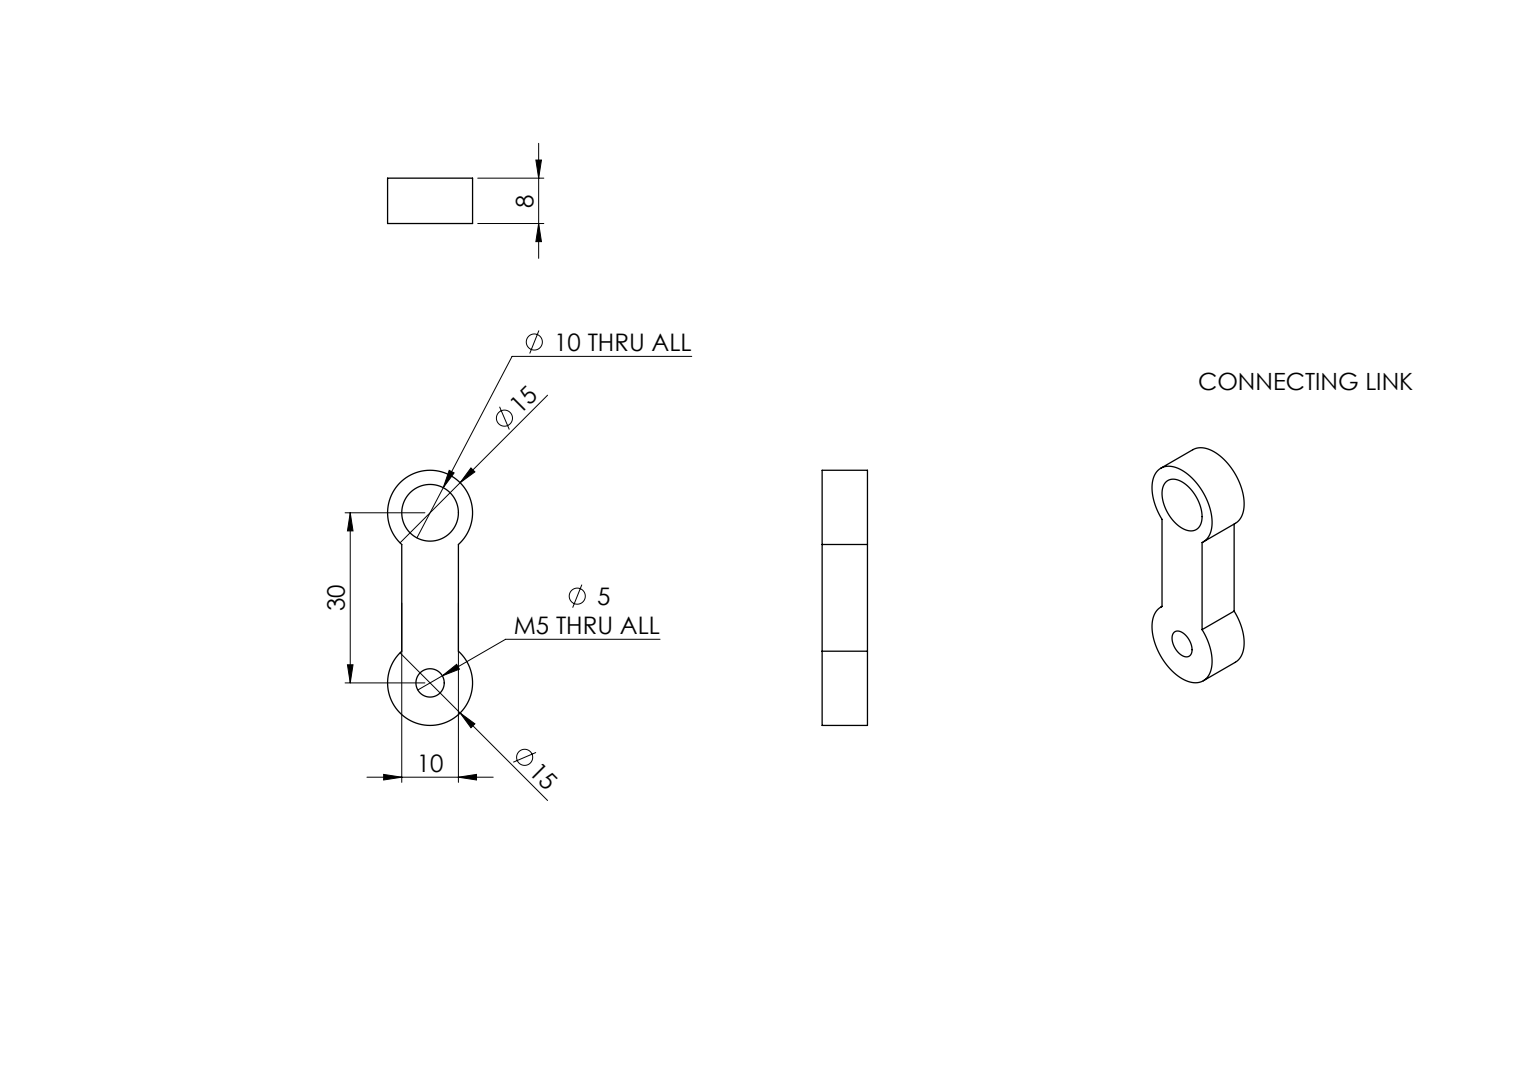
ISO-10303-21;
HEADER;
FILE_DESCRIPTION (('STEP AP214'),
    '1' );
FILE_NAME ('connecting link.step',
    '2026-10-25T11:00:22',
    ( '' ),
    ( '' ),
    'SwSTEP 2.0',
    'SolidWorks 2026',
    '' );
FILE_SCHEMA (( 'AUTOMOTIVE_DESIGN' ));
ENDSEC;

DATA;
#10=DIRECTION ( 'NONE',  ( -1.000000000000000000, 0.000000000000000000, 0.000000000000000000 ) ) ;
#19=CARTESIAN_POINT ( 'NONE',  ( -5.000000000000000000, 5.590169943749474513, 10.00000000000000000 ) ) ;
#25=CYLINDRICAL_SURFACE ( 'NONE', #3173, 4.999999999999999112 ) ;
#27=DIRECTION ( 'NONE',  ( -0.000000000000000000, -0.000000000000000000, -1.000000000000000000 ) ) ;
#30=( LENGTH_UNIT ( ) NAMED_UNIT ( * ) SI_UNIT ( .MILLI., .METRE. ) );
#32=DIRECTION ( 'NONE',  ( -0.000000000000000000, -0.000000000000000000, -1.000000000000000000 ) ) ;
#36=EDGE_CURVE ( 'NONE', #2171, #1853, #1673, .T. ) ;
#37=CIRCLE ( 'NONE', #1306, 7.500000000000000000 ) ;
#58=ORIENTED_EDGE ( 'NONE', *, *, #3093, .T. ) ;
#60=CARTESIAN_POINT ( 'NONE',  ( 4.999999999999999112, 30.00000000000000000, 18.00000000000000355 ) ) ;
#71=CARTESIAN_POINT ( 'NONE',  ( -7.500000000000000000, 0.000000000000000000, 10.00000000000000000 ) ) ;
#73=CARTESIAN_POINT ( 'NONE',  ( 5.000000000000000000, 24.40983005625052726, 18.00000000000000355 ) ) ;
#75=( LENGTH_UNIT ( ) NAMED_UNIT ( * ) SI_UNIT ( .MILLI., .METRE. ) );
#88=ORIENTED_EDGE ( 'NONE', *, *, #36, .T. ) ;
#95=DIRECTION ( 'NONE',  ( -0.000000000000000000, 0.000000000000000000, 1.000000000000000000 ) ) ;
#106=AXIS2_PLACEMENT_3D ( 'NONE', #3179, #664, #3192 ) ;
#113=DIRECTION ( 'NONE',  ( 1.000000000000000000, 0.000000000000000000, 0.000000000000000000 ) ) ;
#125=ORIENTED_EDGE ( 'NONE', *, *, #751, .F. ) ;
#136=EDGE_CURVE ( 'NONE', #870, #2195, #2997, .T. ) ;
#138=AXIS2_PLACEMENT_3D ( 'NONE', #166, #181, #437 ) ;
#146=DIRECTION ( 'NONE',  ( -0.000000000000000000, -0.000000000000000000, -1.000000000000000000 ) ) ;
#152=AXIS2_PLACEMENT_3D ( 'NONE', #2297, #2784, #10 ) ;
#153=CYLINDRICAL_SURFACE ( 'NONE', #3180, 2.499999999999999556 ) ;
#161=EDGE_CURVE ( 'NONE', #1969, #1853, #1067, .T. ) ;
#166=CARTESIAN_POINT ( 'NONE',  ( 0.000000000000000000, 30.00000000000000000, 18.00000000000000355 ) ) ;
#181=DIRECTION ( 'NONE',  ( -0.000000000000000000, -0.000000000000000000, -1.000000000000000000 ) ) ;
#199=ORIENTED_EDGE ( 'NONE', *, *, #2749, .T. ) ;
#207=DIRECTION ( 'NONE',  ( 1.000000000000000000, 0.000000000000000000, 0.000000000000000000 ) ) ;
#222=DIRECTION ( 'NONE',  ( -0.000000000000000000, -0.000000000000000000, -1.000000000000000000 ) ) ;
#237=DIRECTION ( 'NONE',  ( 0.000000000000000000, 0.000000000000000000, 1.000000000000000000 ) ) ;
#243=CIRCLE ( 'NONE', #1828, 7.500000000000000888 ) ;
#245=VECTOR ( 'NONE', #2046, 1000.000000000000000 ) ;
#247=ORIENTED_EDGE ( 'NONE', *, *, #1457, .T. ) ;
#248=AXIS2_PLACEMENT_3D ( 'NONE', #2084, #843, #1137 ) ;
#252=CARTESIAN_POINT ( 'NONE',  ( 0.000000000000000000, 0.000000000000000000, 18.00000000000000355 ) ) ;
#256=SURFACE_SIDE_STYLE ('',( #1538 ) ) ;
#271=FACE_OUTER_BOUND ( 'NONE', #2659, .T. ) ;
#278=( NAMED_UNIT ( * ) PLANE_ANGLE_UNIT ( ) SI_UNIT ( $, .RADIAN. ) );
#280=ADVANCED_FACE ( 'NONE', ( #1859 ), #1120, .F. ) ;
#282=CARTESIAN_POINT ( 'NONE',  ( -7.500000000000000888, 30.00000000000000000, 18.00000000000000355 ) ) ;
#283=ORIENTED_EDGE ( 'NONE', *, *, #618, .F. ) ;
#300=ORIENTED_EDGE ( 'NONE', *, *, #804, .T. ) ;
#303=EDGE_CURVE ( 'NONE', #1969, #1046, #611, .T. ) ;
#310=CARTESIAN_POINT ( 'NONE',  ( 5.000000000000000000, 5.590169943749473624, 10.00000000000000178 ) ) ;
#312=EDGE_LOOP ( 'NONE', ( #1653, #125 ) ) ;
#313=LINE ( 'NONE', #1936, #1957 ) ;
#314=AXIS2_PLACEMENT_3D ( 'NONE', #858, #1399, #2660 ) ;
#317=ORIENTED_EDGE ( 'NONE', *, *, #2514, .F. ) ;
#327=FILL_AREA_STYLE ('',( #2835 ) ) ;
#334=CARTESIAN_POINT ( 'NONE',  ( -4.999999999999999112, 30.00000000000000000, 18.00000000000000355 ) ) ;
#338=ORIENTED_EDGE ( 'NONE', *, *, #2208, .F. ) ;
#342=VERTEX_POINT ( 'NONE', #19 ) ;
#347=EDGE_CURVE ( 'NONE', #1810, #870, #2221, .T. ) ;
#352=EDGE_LOOP ( 'NONE', ( #2643, #317, #2086, #589 ) ) ;
#357=PRODUCT ( 'connecting link', 'connecting link', '', ( #2766 ) ) ;
#362=EDGE_CURVE ( 'NONE', #342, #3130, #37, .T. ) ;
#371=AXIS2_PLACEMENT_3D ( 'NONE', #462, #759, #1502 ) ;
#376=ORIENTED_EDGE ( 'NONE', *, *, #347, .F. ) ;
#380=ORIENTED_EDGE ( 'NONE', *, *, #362, .T. ) ;
#409=ORIENTED_EDGE ( 'NONE', *, *, #362, .F. ) ;
#431=MECHANICAL_DESIGN_GEOMETRIC_PRESENTATION_REPRESENTATION('',(#1645),#485);
#437=DIRECTION ( 'NONE',  ( -1.000000000000000000, 0.000000000000000000, 0.000000000000000000 ) ) ;
#439=VERTEX_POINT ( 'NONE', #282 ) ;
#445=DIRECTION ( 'NONE',  ( 1.000000000000000000, 0.000000000000000000, 0.000000000000000000 ) ) ;
#447=CARTESIAN_POINT ( 'NONE',  ( -2.499999999999999556, 3.061616997868382648E-16, 10.00000000000000000 ) ) ;
#462=CARTESIAN_POINT ( 'NONE',  ( 0.000000000000000000, 30.00000000000000000, 18.00000000000000355 ) ) ;
#464=EDGE_CURVE ( 'NONE', #1883, #2883, #2843, .T. ) ;
#469=CARTESIAN_POINT ( 'NONE',  ( 0.000000000000000000, 30.00000000000000000, 18.00000000000000355 ) ) ;
#475=CARTESIAN_POINT ( 'NONE',  ( 0.000000000000000000, 30.00000000000000000, 10.00000000000000000 ) ) ;
#478=DIRECTION ( 'NONE',  ( 1.000000000000000000, 0.000000000000000000, 0.000000000000000000 ) ) ;
#485=( GEOMETRIC_REPRESENTATION_CONTEXT ( 3 ) GLOBAL_UNCERTAINTY_ASSIGNED_CONTEXT ( ( #770 ) ) GLOBAL_UNIT_ASSIGNED_CONTEXT ( ( #75, #3051, #1811 ) ) REPRESENTATION_CONTEXT ( 'NONE', 'WORKASPACE' ) );
#488=ORIENTED_EDGE ( 'NONE', *, *, #2125, .F. ) ;
#500=EDGE_LOOP ( 'NONE', ( #2350, #616 ) ) ;
#508=LINE ( 'NONE', #2045, #3059 ) ;
#520=EDGE_LOOP ( 'NONE', ( #2673, #606, #711, #2356 ) ) ;
#548=LINE ( 'NONE', #2266, #1038 ) ;
#558=EDGE_CURVE ( 'NONE', #1156, #900, #2476, .T. ) ;
#560=ORIENTED_EDGE ( 'NONE', *, *, #1874, .F. ) ;
#561=DIRECTION ( 'NONE',  ( 1.000000000000000000, 0.000000000000000000, 0.000000000000000000 ) ) ;
#563=EDGE_LOOP ( 'NONE', ( #962, #2420, #624, #283 ) ) ;
#567=ORIENTED_EDGE ( 'NONE', *, *, #2749, .F. ) ;
#576=EDGE_LOOP ( 'NONE', ( #2530, #2251, #199, #247, #1827, #3157, #1316, #88 ) ) ;
#578=CARTESIAN_POINT ( 'NONE',  ( 0.000000000000000000, 30.00000000000000000, 18.00000000000000355 ) ) ;
#582=ORIENTED_EDGE ( 'NONE', *, *, #2260, .F. ) ;
#583=AXIS2_PLACEMENT_3D ( 'NONE', #2757, #3243, #478 ) ;
#585=VECTOR ( 'NONE', #739, 1000.000000000000000 ) ;
#589=ORIENTED_EDGE ( 'NONE', *, *, #2208, .T. ) ;
#595=CARTESIAN_POINT ( 'NONE',  ( 0.000000000000000000, 0.000000000000000000, 10.00000000000000000 ) ) ;
#599=DIRECTION ( 'NONE',  ( -1.000000000000000000, 0.000000000000000000, -0.000000000000000000 ) ) ;
#606=ORIENTED_EDGE ( 'NONE', *, *, #161, .T. ) ;
#611=LINE ( 'NONE', #73, #1572 ) ;
#616=ORIENTED_EDGE ( 'NONE', *, *, #136, .F. ) ;
#617=ADVANCED_BREP_SHAPE_REPRESENTATION ( '', ( #1595, #1692 ), #2651 ) ;
#618=EDGE_CURVE ( 'NONE', #1320, #3085, #548, .T. ) ;
#624=ORIENTED_EDGE ( 'NONE', *, *, #2822, .T. ) ;
#630=VECTOR ( 'NONE', #32, 1000.000000000000000 ) ;
#631=ORIENTED_EDGE ( 'NONE', *, *, #2234, .F. ) ;
#636=ADVANCED_FACE ( 'NONE', ( #1251 ), #2803, .F. ) ;
#642=AXIS2_PLACEMENT_3D ( 'NONE', #1934, #2512, #954 ) ;
#652=ADVANCED_FACE ( 'NONE', ( #1812, #1779, #2515 ), #3022, .T. ) ;
#664=DIRECTION ( 'NONE',  ( -0.000000000000000000, -0.000000000000000000, 1.000000000000000000 ) ) ;
#670=DIRECTION ( 'NONE',  ( 0.000000000000000000, 0.000000000000000000, 1.000000000000000000 ) ) ;
#676=DIRECTION ( 'NONE',  ( -0.000000000000000000, -0.000000000000000000, -1.000000000000000000 ) ) ;
#694=VERTEX_POINT ( 'NONE', #2035 ) ;
#696=CARTESIAN_POINT ( 'NONE',  ( 0.000000000000000000, 30.00000000000000000, 18.00000000000000355 ) ) ;
#699=LINE ( 'NONE', #985, #1260 ) ;
#708=CARTESIAN_POINT ( 'NONE',  ( 0.000000000000000000, 30.00000000000000000, 18.00000000000000355 ) ) ;
#711=ORIENTED_EDGE ( 'NONE', *, *, #1884, .T. ) ;
#716=DIRECTION ( 'NONE',  ( -1.000000000000000000, 0.000000000000000000, 0.000000000000000000 ) ) ;
#723=DIRECTION ( 'NONE',  ( -0.000000000000000000, -0.000000000000000000, -1.000000000000000000 ) ) ;
#725=DIRECTION ( 'NONE',  ( 1.000000000000000000, 0.000000000000000000, 0.000000000000000000 ) ) ;
#737=ORIENTED_EDGE ( 'NONE', *, *, #2840, .T. ) ;
#739=DIRECTION ( 'NONE',  ( -0.000000000000000000, -0.000000000000000000, 1.000000000000000000 ) ) ;
#742=CIRCLE ( 'NONE', #2590, 2.499999999999999556 ) ;
#743=FACE_BOUND ( 'NONE', #2335, .T. ) ;
#751=EDGE_CURVE ( 'NONE', #2182, #2708, #3107, .T. ) ;
#753=ORIENTED_EDGE ( 'NONE', *, *, #2111, .F. ) ;
#759=DIRECTION ( 'NONE',  ( 0.000000000000000000, 0.000000000000000000, 1.000000000000000000 ) ) ;
#768=CARTESIAN_POINT ( 'NONE',  ( 0.000000000000000000, 0.000000000000000000, 18.00000000000000355 ) ) ;
#770=UNCERTAINTY_MEASURE_WITH_UNIT (LENGTH_MEASURE( 1.000000000000000082E-05 ), #75, 'distance_accuracy_value', 'NONE');
#781=DIRECTION ( 'NONE',  ( -0.000000000000000000, -0.000000000000000000, 1.000000000000000000 ) ) ;
#789=DIRECTION ( 'NONE',  ( -0.000000000000000000, -0.000000000000000000, 1.000000000000000000 ) ) ;
#790=CARTESIAN_POINT ( 'NONE',  ( 0.000000000000000000, 30.00000000000000000, 18.00000000000000355 ) ) ;
#799=ORIENTED_EDGE ( 'NONE', *, *, #2840, .F. ) ;
#804=EDGE_CURVE ( 'NONE', #694, #2199, #2047, .T. ) ;
#808=DIRECTION ( 'NONE',  ( 1.000000000000000000, 0.000000000000000000, -0.000000000000000000 ) ) ;
#837=EDGE_CURVE ( 'NONE', #2412, #2195, #3144, .T. ) ;
#843=DIRECTION ( 'NONE',  ( -0.000000000000000000, -0.000000000000000000, 1.000000000000000000 ) ) ;
#847=CARTESIAN_POINT ( 'NONE',  ( -4.999999999999998224, 30.00000000000000000, 10.00000000000000000 ) ) ;
#856=PRODUCT_DEFINITION_FORMATION_WITH_SPECIFIED_SOURCE ( 'ANY', '', #357, .NOT_KNOWN. ) ;
#858=CARTESIAN_POINT ( 'NONE',  ( 0.000000000000000000, 30.00000000000000000, 10.00000000000000000 ) ) ;
#859=DIRECTION ( 'NONE',  ( 1.000000000000000000, 0.000000000000000000, 0.000000000000000000 ) ) ;
#865=ORIENTED_EDGE ( 'NONE', *, *, #2062, .F. ) ;
#870=VERTEX_POINT ( 'NONE', #2333 ) ;
#878=ORIENTED_EDGE ( 'NONE', *, *, #2178, .F. ) ;
#886=PRODUCT_DEFINITION_SHAPE ( 'NONE', 'NONE',  #3057 ) ;
#893=ORIENTED_EDGE ( 'NONE', *, *, #2988, .F. ) ;
#900=VERTEX_POINT ( 'NONE', #310 ) ;
#915=DIRECTION ( 'NONE',  ( -1.000000000000000000, 0.000000000000000000, 0.000000000000000000 ) ) ;
#928=ORIENTED_EDGE ( 'NONE', *, *, #837, .T. ) ;
#933=EDGE_LOOP ( 'NONE', ( #1125, #878, #1413, #2404 ) ) ;
#934=DIRECTION ( 'NONE',  ( 1.000000000000000000, 0.000000000000000000, 0.000000000000000000 ) ) ;
#945=AXIS2_PLACEMENT_3D ( 'NONE', #2977, #2731, #716 ) ;
#949=ORIENTED_EDGE ( 'NONE', *, *, #2612, .T. ) ;
#951=CARTESIAN_POINT ( 'NONE',  ( -5.000000000000000000, 30.00000000000000000, 10.00000000000000178 ) ) ;
#954=DIRECTION ( 'NONE',  ( 1.000000000000000000, 0.000000000000000000, 0.000000000000000000 ) ) ;
#962=ORIENTED_EDGE ( 'NONE', *, *, #1457, .F. ) ;
#970=LINE ( 'NONE', #1953, #1479 ) ;
#978=ADVANCED_FACE ( 'NONE', ( #3108 ), #2402, .T. ) ;
#982=STYLED_ITEM('',(#3300),#1595);
#985=CARTESIAN_POINT ( 'NONE',  ( 5.000000000000000000, 30.00000000000000000, 10.00000000000000178 ) ) ;
#989=DIRECTION ( 'NONE',  ( -1.000000000000000000, 0.000000000000000000, -0.000000000000000000 ) ) ;
#997=CARTESIAN_POINT ( 'NONE',  ( -7.500000000000000000, 0.000000000000000000, 18.00000000000000355 ) ) ;
#1001=PRODUCT_DEFINITION_CONTEXT ( 'detailed design', #2486, 'design' ) ;
#1009=ORIENTED_EDGE ( 'NONE', *, *, #2612, .F. ) ;
#1016=CARTESIAN_POINT ( 'NONE',  ( -5.000000000000000000, 5.590169943749474513, 18.00000000000000355 ) ) ;
#1022=CARTESIAN_POINT ( 'NONE',  ( -5.000000000000000000, 5.590169943749473624, 18.00000000000000355 ) ) ;
#1025=DIRECTION ( 'NONE',  ( -0.000000000000000000, -0.000000000000000000, 1.000000000000000000 ) ) ;
#1030=FACE_OUTER_BOUND ( 'NONE', #1593, .T. ) ;
#1031=CARTESIAN_POINT ( 'NONE',  ( 0.000000000000000000, 30.00000000000000000, 18.00000000000000355 ) ) ;
#1032=CARTESIAN_POINT ( 'NONE',  ( 5.000000000000000000, 30.00000000000000000, 18.00000000000000355 ) ) ;
#1038=VECTOR ( 'NONE', #27, 1000.000000000000000 ) ;
#1046=VERTEX_POINT ( 'NONE', #1951 ) ;
#1051=DIRECTION ( 'NONE',  ( 1.000000000000000000, 0.000000000000000000, 0.000000000000000000 ) ) ;
#1060=CARTESIAN_POINT ( 'NONE',  ( 0.000000000000000000, 0.000000000000000000, 10.00000000000000000 ) ) ;
#1067=LINE ( 'NONE', #1032, #245 ) ;
#1087=VERTEX_POINT ( 'NONE', #2290 ) ;
#1098=AXIS2_PLACEMENT_3D ( 'NONE', #2889, #2386, #113 ) ;
#1105=VECTOR ( 'NONE', #146, 1000.000000000000000 ) ;
#1120=CYLINDRICAL_SURFACE ( 'NONE', #2368, 4.999999999999999112 ) ;
#1122=CARTESIAN_POINT ( 'NONE',  ( 2.500000000000000000, 0.000000000000000000, 18.00000000000000355 ) ) ;
#1125=ORIENTED_EDGE ( 'NONE', *, *, #464, .F. ) ;
#1137=DIRECTION ( 'NONE',  ( 1.000000000000000000, 0.000000000000000000, 0.000000000000000000 ) ) ;
#1156=VERTEX_POINT ( 'NONE', #2322 ) ;
#1162=AXIS2_PLACEMENT_3D ( 'NONE', #768, #2279, #2755 ) ;
#1180=ORIENTED_EDGE ( 'NONE', *, *, #837, .F. ) ;
#1197=( GEOMETRIC_REPRESENTATION_CONTEXT ( 3 ) GLOBAL_UNCERTAINTY_ASSIGNED_CONTEXT ( ( #3048 ) ) GLOBAL_UNIT_ASSIGNED_CONTEXT ( ( #30, #278, #3056 ) ) REPRESENTATION_CONTEXT ( 'NONE', 'WORKASPACE' ) );
#1200=ORIENTED_EDGE ( 'NONE', *, *, #2712, .F. ) ;
#1206=CARTESIAN_POINT ( 'NONE',  ( 7.500000000000000888, 30.00000000000000000, 18.00000000000000355 ) ) ;
#1208=CARTESIAN_POINT ( 'NONE',  ( 0.000000000000000000, 0.000000000000000000, 10.00000000000000000 ) ) ;
#1212=AXIS2_PLACEMENT_3D ( 'NONE', #1488, #1986, #1731 ) ;
#1220=DIRECTION ( 'NONE',  ( -1.000000000000000000, 0.000000000000000000, 0.000000000000000000 ) ) ;
#1221=DIRECTION ( 'NONE',  ( 0.000000000000000000, 0.000000000000000000, 1.000000000000000000 ) ) ;
#1236=SHAPE_REPRESENTATION ( 'connecting link', ( #1692 ), #2651 ) ;
#1242=ORIENTED_EDGE ( 'NONE', *, *, #558, .F. ) ;
#1248=VECTOR ( 'NONE', #2015, 1000.000000000000000 ) ;
#1251=FACE_OUTER_BOUND ( 'NONE', #520, .T. ) ;
#1257=ORIENTED_EDGE ( 'NONE', *, *, #2988, .T. ) ;
#1260=VECTOR ( 'NONE', #1699, 1000.000000000000000 ) ;
#1267=CARTESIAN_POINT ( 'NONE',  ( 0.000000000000000000, 0.000000000000000000, 18.00000000000000355 ) ) ;
#1272=EDGE_CURVE ( 'NONE', #2870, #3130, #3268, .T. ) ;
#1280=FACE_OUTER_BOUND ( 'NONE', #3189, .T. ) ;
#1306=AXIS2_PLACEMENT_3D ( 'NONE', #1060, #2108, #3115 ) ;
#1315=DIRECTION ( 'NONE',  ( -0.000000000000000000, -0.000000000000000000, 1.000000000000000000 ) ) ;
#1316=ORIENTED_EDGE ( 'NONE', *, *, #2514, .T. ) ;
#1320=VERTEX_POINT ( 'NONE', #1394 ) ;
#1322=AXIS2_PLACEMENT_3D ( 'NONE', #708, #781, #2215 ) ;
#1331=DIRECTION ( 'NONE',  ( -0.000000000000000000, -0.000000000000000000, 1.000000000000000000 ) ) ;
#1336=ORIENTED_EDGE ( 'NONE', *, *, #2260, .T. ) ;
#1375=AXIS2_PLACEMENT_3D ( 'NONE', #2936, #2973, #934 ) ;
#1385=CARTESIAN_POINT ( 'NONE',  ( 2.499999999999999556, 0.000000000000000000, 18.00000000000000355 ) ) ;
#1394=CARTESIAN_POINT ( 'NONE',  ( -5.000000000000000000, 24.40983005625052726, 18.00000000000000355 ) ) ;
#1399=DIRECTION ( 'NONE',  ( 0.000000000000000000, 0.000000000000000000, 1.000000000000000000 ) ) ;
#1411=MECHANICAL_DESIGN_GEOMETRIC_PRESENTATION_REPRESENTATION('',(#982),#1197);
#1413=ORIENTED_EDGE ( 'NONE', *, *, #303, .T. ) ;
#1415=CARTESIAN_POINT ( 'NONE',  ( 0.000000000000000000, 0.000000000000000000, 18.00000000000000355 ) ) ;
#1424=AXIS2_PLACEMENT_3D ( 'NONE', #3226, #237, #207 ) ;
#1449=LINE ( 'NONE', #951, #2117 ) ;
#1451=DIRECTION ( 'NONE',  ( -0.000000000000000000, -0.000000000000000000, -1.000000000000000000 ) ) ;
#1453=LINE ( 'NONE', #2174, #1105 ) ;
#1457=EDGE_CURVE ( 'NONE', #439, #1320, #243, .T. ) ;
#1465=APPLICATION_CONTEXT ( 'automotive_design' ) ;
#1469=CARTESIAN_POINT ( 'NONE',  ( -2.500000000000000000, 3.061616997868383141E-16, 18.00000000000000355 ) ) ;
#1479=VECTOR ( 'NONE', #1451, 1000.000000000000000 ) ;
#1485=DIRECTION ( 'NONE',  ( 0.000000000000000000, 1.000000000000000000, 0.000000000000000000 ) ) ;
#1488=CARTESIAN_POINT ( 'NONE',  ( 0.000000000000000000, 0.000000000000000000, 10.00000000000000000 ) ) ;
#1495=ADVANCED_FACE ( 'NONE', ( #2706 ), #2687, .T. ) ;
#1502=DIRECTION ( 'NONE',  ( 1.000000000000000000, 0.000000000000000000, 0.000000000000000000 ) ) ;
#1514=DIRECTION ( 'NONE',  ( -0.000000000000000000, -1.000000000000000000, 0.000000000000000000 ) ) ;
#1522=ORIENTED_EDGE ( 'NONE', *, *, #2781, .T. ) ;
#1526=ORIENTED_EDGE ( 'NONE', *, *, #3093, .F. ) ;
#1538=SURFACE_STYLE_FILL_AREA ( #327 ) ;
#1565=PRESENTATION_STYLE_ASSIGNMENT (( #2332 ) ) ;
#1571=CARTESIAN_POINT ( 'NONE',  ( 5.000000000000000000, 5.590169943749473624, 18.00000000000000355 ) ) ;
#1572=VECTOR ( 'NONE', #1841, 1000.000000000000000 ) ;
#1593=EDGE_LOOP ( 'NONE', ( #1526, #949, #2318, #1200 ) ) ;
#1595=MANIFOLD_SOLID_BREP ( 'AdvancedHole1', #2472 ) ;
#1608=LINE ( 'NONE', #2624, #585 ) ;
#1610=ORIENTED_EDGE ( 'NONE', *, *, #2781, .F. ) ;
#1616=DIRECTION ( 'NONE',  ( -0.000000000000000000, -0.000000000000000000, 1.000000000000000000 ) ) ;
#1639=CIRCLE ( 'NONE', #314, 7.500000000000000888 ) ;
#1645=STYLED_ITEM ( 'NONE', ( #1565 ), #617 ) ;
#1653=ORIENTED_EDGE ( 'NONE', *, *, #2059, .F. ) ;
#1673=CIRCLE ( 'NONE', #3159, 7.500000000000000000 ) ;
#1685=DIRECTION ( 'NONE',  ( -0.000000000000000000, -0.000000000000000000, -1.000000000000000000 ) ) ;
#1689=DIRECTION ( 'NONE',  ( 1.000000000000000000, 0.000000000000000000, 0.000000000000000000 ) ) ;
#1690=AXIS2_PLACEMENT_3D ( 'NONE', #1984, #2956, #445 ) ;
#1692=AXIS2_PLACEMENT_3D ( 'NONE', #3075, #2051, #2104 ) ;
#1699=DIRECTION ( 'NONE',  ( 0.000000000000000000, 1.000000000000000000, 0.000000000000000000 ) ) ;
#1726=CYLINDRICAL_SURFACE ( 'NONE', #2593, 7.500000000000000000 ) ;
#1731=DIRECTION ( 'NONE',  ( 1.000000000000000000, 0.000000000000000000, -0.000000000000000000 ) ) ;
#1740=CIRCLE ( 'NONE', #106, 2.500000000000000000 ) ;
#1760=DIRECTION ( 'NONE',  ( -0.000000000000000000, -0.000000000000000000, 1.000000000000000000 ) ) ;
#1761=UNCERTAINTY_MEASURE_WITH_UNIT (LENGTH_MEASURE( 1.000000000000000082E-05 ), #2666, 'distance_accuracy_value', 'NONE');
#1769=ORIENTED_EDGE ( 'NONE', *, *, #2712, .T. ) ;
#1779=FACE_BOUND ( 'NONE', #500, .T. ) ;
#1785=CARTESIAN_POINT ( 'NONE',  ( 7.500000000000000888, 30.00000000000000000, 18.00000000000000355 ) ) ;
#1790=CIRCLE ( 'NONE', #371, 7.500000000000000888 ) ;
#1793=CIRCLE ( 'NONE', #1690, 7.500000000000000888 ) ;
#1797=CARTESIAN_POINT ( 'NONE',  ( 5.000000000000000000, 30.00000000000000000, -21.62277660168378901 ) ) ;
#1803=ORIENTED_EDGE ( 'NONE', *, *, #347, .T. ) ;
#1810=VERTEX_POINT ( 'NONE', #847 ) ;
#1811=( NAMED_UNIT ( * ) SI_UNIT ( $, .STERADIAN. ) SOLID_ANGLE_UNIT ( ) );
#1812=FACE_BOUND ( 'NONE', #312, .T. ) ;
#1823=ORIENTED_EDGE ( 'NONE', *, *, #2062, .T. ) ;
#1827=ORIENTED_EDGE ( 'NONE', *, *, #2234, .T. ) ;
#1828=AXIS2_PLACEMENT_3D ( 'NONE', #469, #670, #1689 ) ;
#1841=DIRECTION ( 'NONE',  ( -0.000000000000000000, -0.000000000000000000, -1.000000000000000000 ) ) ;
#1853=VERTEX_POINT ( 'NONE', #1571 ) ;
#1859=FACE_OUTER_BOUND ( 'NONE', #2664, .T. ) ;
#1874=EDGE_CURVE ( 'NONE', #439, #1087, #313, .T. ) ;
#1883=VERTEX_POINT ( 'NONE', #1206 ) ;
#1884=EDGE_CURVE ( 'NONE', #1853, #900, #1453, .T. ) ;
#1894=CARTESIAN_POINT ( 'NONE',  ( -5.000000000000000000, 24.40983005625052726, 10.00000000000000178 ) ) ;
#1902=VECTOR ( 'NONE', #2033, 1000.000000000000000 ) ;
#1913=ADVANCED_FACE ( 'NONE', ( #3209 ), #1955, .T. ) ;
#1914=ORIENTED_EDGE ( 'NONE', *, *, #618, .T. ) ;
#1918=ORIENTED_EDGE ( 'NONE', *, *, #2868, .F. ) ;
#1929=CARTESIAN_POINT ( 'NONE',  ( 0.000000000000000000, 0.000000000000000000, 18.00000000000000355 ) ) ;
#1931=ORIENTED_EDGE ( 'NONE', *, *, #1272, .F. ) ;
#1934=CARTESIAN_POINT ( 'NONE',  ( 0.000000000000000000, 30.00000000000000000, 10.00000000000000000 ) ) ;
#1936=CARTESIAN_POINT ( 'NONE',  ( -7.500000000000000888, 30.00000000000000000, 18.00000000000000355 ) ) ;
#1951=CARTESIAN_POINT ( 'NONE',  ( 5.000000000000000000, 24.40983005625052726, 10.00000000000000178 ) ) ;
#1953=CARTESIAN_POINT ( 'NONE',  ( 7.500000000000000000, 9.184850993605147944E-16, 18.00000000000000355 ) ) ;
#1955=CYLINDRICAL_SURFACE ( 'NONE', #945, 7.500000000000000000 ) ;
#1957=VECTOR ( 'NONE', #1685, 1000.000000000000000 ) ;
#1963=EDGE_LOOP ( 'NONE', ( #631, #1914, #799, #582 ) ) ;
#1966=DIRECTION ( 'NONE',  ( 1.000000000000000000, 0.000000000000000000, 0.000000000000000000 ) ) ;
#1969=VERTEX_POINT ( 'NONE', #2153 ) ;
#1984=CARTESIAN_POINT ( 'NONE',  ( 0.000000000000000000, 30.00000000000000000, 10.00000000000000000 ) ) ;
#1986=DIRECTION ( 'NONE',  ( 0.000000000000000000, 0.000000000000000000, 1.000000000000000000 ) ) ;
#2005=DIRECTION ( 'NONE',  ( -0.000000000000000000, 0.000000000000000000, 1.000000000000000000 ) ) ;
#2014=AXIS2_PLACEMENT_3D ( 'NONE', #475, #2987, #2235 ) ;
#2015=DIRECTION ( 'NONE',  ( -0.000000000000000000, -0.000000000000000000, -1.000000000000000000 ) ) ;
#2033=DIRECTION ( 'NONE',  ( -0.000000000000000000, -0.000000000000000000, -1.000000000000000000 ) ) ;
#2035=CARTESIAN_POINT ( 'NONE',  ( 2.499999999999999556, 0.000000000000000000, 10.00000000000000000 ) ) ;
#2045=CARTESIAN_POINT ( 'NONE',  ( -5.000000000000000000, 30.00000000000000000, 18.00000000000000355 ) ) ;
#2046=DIRECTION ( 'NONE',  ( -0.000000000000000000, -1.000000000000000000, 0.000000000000000000 ) ) ;
#2047=CIRCLE ( 'NONE', #1098, 2.499999999999999556 ) ;
#2051=DIRECTION ( 'NONE',  ( 0.000000000000000000, 0.000000000000000000, 1.000000000000000000 ) ) ;
#2059=EDGE_CURVE ( 'NONE', #2708, #2182, #1740, .T. ) ;
#2062=EDGE_CURVE ( 'NONE', #1810, #2412, #2269, .T. ) ;
#2084=CARTESIAN_POINT ( 'NONE',  ( 0.000000000000000000, 0.000000000000000000, 18.00000000000000355 ) ) ;
#2086=ORIENTED_EDGE ( 'NONE', *, *, #1272, .T. ) ;
#2096=AXIS2_PLACEMENT_3D ( 'NONE', #2857, #599, #95 ) ;
#2104=DIRECTION ( 'NONE',  ( 1.000000000000000000, 0.000000000000000000, 0.000000000000000000 ) ) ;
#2108=DIRECTION ( 'NONE',  ( 0.000000000000000000, 0.000000000000000000, 1.000000000000000000 ) ) ;
#2111=EDGE_CURVE ( 'NONE', #900, #1046, #699, .T. ) ;
#2114=AXIS2_PLACEMENT_3D ( 'NONE', #2990, #222, #1220 ) ;
#2117=VECTOR ( 'NONE', #1485, 1000.000000000000000 ) ;
#2119=DIRECTION ( 'NONE',  ( -0.000000000000000000, -0.000000000000000000, 1.000000000000000000 ) ) ;
#2125=EDGE_CURVE ( 'NONE', #3214, #2870, #3007, .T. ) ;
#2136=EDGE_LOOP ( 'NONE', ( #300, #58 ) ) ;
#2137=LINE ( 'NONE', #1385, #2227 ) ;
#2140=ORIENTED_EDGE ( 'NONE', *, *, #464, .T. ) ;
#2149=ADVANCED_FACE ( 'NONE', ( #2975, #743, #3273 ), #3256, .F. ) ;
#2150=ORIENTED_EDGE ( 'NONE', *, *, #2822, .F. ) ;
#2153=CARTESIAN_POINT ( 'NONE',  ( 5.000000000000000000, 24.40983005625052726, 18.00000000000000355 ) ) ;
#2165=ADVANCED_FACE ( 'NONE', ( #3207 ), #2450, .T. ) ;
#2171=VERTEX_POINT ( 'NONE', #2729 ) ;
#2174=CARTESIAN_POINT ( 'NONE',  ( 5.000000000000000000, 5.590169943749474513, 18.00000000000000355 ) ) ;
#2178=EDGE_CURVE ( 'NONE', #1969, #1883, #1790, .T. ) ;
#2182=VERTEX_POINT ( 'NONE', #1469 ) ;
#2195=VERTEX_POINT ( 'NONE', #2237 ) ;
#2197=CYLINDRICAL_SURFACE ( 'NONE', #2752, 7.500000000000000000 ) ;
#2198=CARTESIAN_POINT ( 'NONE',  ( 4.999999999999998224, 30.00000000000000000, 10.00000000000000000 ) ) ;
#2199=VERTEX_POINT ( 'NONE', #447 ) ;
#2208=EDGE_CURVE ( 'NONE', #3130, #1156, #3119, .T. ) ;
#2213=EDGE_CURVE ( 'NONE', #2171, #1156, #970, .T. ) ;
#2215=DIRECTION ( 'NONE',  ( 1.000000000000000000, 0.000000000000000000, 0.000000000000000000 ) ) ;
#2221=LINE ( 'NONE', #334, #2678 ) ;
#2227=VECTOR ( 'NONE', #2401, 1000.000000000000000 ) ;
#2234=EDGE_CURVE ( 'NONE', #1320, #3214, #508, .T. ) ;
#2235=DIRECTION ( 'NONE',  ( 1.000000000000000000, 0.000000000000000000, 0.000000000000000000 ) ) ;
#2237=CARTESIAN_POINT ( 'NONE',  ( 4.999999999999999112, 30.00000000000000000, 18.00000000000000355 ) ) ;
#2247=ADVANCED_FACE ( 'NONE', ( #271 ), #2282, .T. ) ;
#2251=ORIENTED_EDGE ( 'NONE', *, *, #2178, .T. ) ;
#2260=EDGE_CURVE ( 'NONE', #3214, #342, #3031, .T. ) ;
#2266=CARTESIAN_POINT ( 'NONE',  ( -5.000000000000000000, 24.40983005625052726, 18.00000000000000355 ) ) ;
#2269=CIRCLE ( 'NONE', #642, 4.999999999999998224 ) ;
#2279=DIRECTION ( 'NONE',  ( 0.000000000000000000, 0.000000000000000000, 1.000000000000000000 ) ) ;
#2282=CYLINDRICAL_SURFACE ( 'NONE', #152, 7.500000000000000888 ) ;
#2289=CARTESIAN_POINT ( 'NONE',  ( 0.000000000000000000, 0.000000000000000000, 18.00000000000000355 ) ) ;
#2290=CARTESIAN_POINT ( 'NONE',  ( -7.500000000000000888, 30.00000000000000000, 10.00000000000000000 ) ) ;
#2292=ORIENTED_EDGE ( 'NONE', *, *, #136, .T. ) ;
#2297=CARTESIAN_POINT ( 'NONE',  ( 0.000000000000000000, 30.00000000000000000, 18.00000000000000355 ) ) ;
#2315=SHAPE_REPRESENTATION_RELATIONSHIP ( 'NONE' , 'NONE' ,  #1236, #617 ) ;
#2318=ORIENTED_EDGE ( 'NONE', *, *, #751, .T. ) ;
#2321=EDGE_LOOP ( 'NONE', ( #1931, #488, #1336, #380 ) ) ;
#2322=CARTESIAN_POINT ( 'NONE',  ( 7.500000000000000000, 9.184850993605147944E-16, 10.00000000000000000 ) ) ;
#2323=ADVANCED_FACE ( 'NONE', ( #1280 ), #25, .F. ) ;
#2330=DIRECTION ( 'NONE',  ( 1.000000000000000000, 0.000000000000000000, 0.000000000000000000 ) ) ;
#2332=SURFACE_STYLE_USAGE ( .BOTH. , #256 ) ;
#2333=CARTESIAN_POINT ( 'NONE',  ( -4.999999999999999112, 30.00000000000000000, 18.00000000000000355 ) ) ;
#2335=EDGE_LOOP ( 'NONE', ( #1522, #1823 ) ) ;
#2343=ORIENTED_EDGE ( 'NONE', *, *, #804, .F. ) ;
#2350=ORIENTED_EDGE ( 'NONE', *, *, #3241, .F. ) ;
#2356=ORIENTED_EDGE ( 'NONE', *, *, #2111, .T. ) ;
#2367=ORIENTED_EDGE ( 'NONE', *, *, #2059, .T. ) ;
#2368=AXIS2_PLACEMENT_3D ( 'NONE', #578, #1616, #859 ) ;
#2383=CIRCLE ( 'NONE', #2795, 7.500000000000000888 ) ;
#2386=DIRECTION ( 'NONE',  ( -0.000000000000000000, -0.000000000000000000, 1.000000000000000000 ) ) ;
#2401=DIRECTION ( 'NONE',  ( -0.000000000000000000, -0.000000000000000000, 1.000000000000000000 ) ) ;
#2402=PLANE ( 'NONE',  #2096 ) ;
#2404=ORIENTED_EDGE ( 'NONE', *, *, #2868, .T. ) ;
#2412=VERTEX_POINT ( 'NONE', #2198 ) ;
#2413=DIRECTION ( 'NONE',  ( 1.000000000000000000, 0.000000000000000000, 0.000000000000000000 ) ) ;
#2420=ORIENTED_EDGE ( 'NONE', *, *, #1874, .T. ) ;
#2428=FACE_OUTER_BOUND ( 'NONE', #2442, .T. ) ;
#2442=EDGE_LOOP ( 'NONE', ( #1009, #2343, #1769, #2367 ) ) ;
#2446=ORIENTED_EDGE ( 'NONE', *, *, #2213, .T. ) ;
#2450=CYLINDRICAL_SURFACE ( 'NONE', #2114, 7.500000000000000888 ) ;
#2460=EDGE_LOOP ( 'NONE', ( #1918, #753, #1242, #338, #409, #737, #2150, #893 ) ) ;
#2472=CLOSED_SHELL ( 'NONE', ( #2928, #2323, #2247, #1495, #3141, #1913, #636, #978, #3258, #652, #2149, #2165, #280, #2855 ) ) ;
#2476=CIRCLE ( 'NONE', #3259, 7.500000000000000000 ) ;
#2478=FACE_OUTER_BOUND ( 'NONE', #2321, .T. ) ;
#2480=ORIENTED_EDGE ( 'NONE', *, *, #36, .F. ) ;
#2486=APPLICATION_CONTEXT ( 'automotive_design' ) ;
#2493=CIRCLE ( 'NONE', #1322, 4.999999999999999112 ) ;
#2497=CARTESIAN_POINT ( 'NONE',  ( 7.500000000000000888, 30.00000000000000000, 10.00000000000000000 ) ) ;
#2512=DIRECTION ( 'NONE',  ( -0.000000000000000000, -0.000000000000000000, 1.000000000000000000 ) ) ;
#2514=EDGE_CURVE ( 'NONE', #2870, #2171, #2904, .T. ) ;
#2515=FACE_OUTER_BOUND ( 'NONE', #576, .T. ) ;
#2525=AXIS2_PLACEMENT_3D ( 'NONE', #1267, #1221, #808 ) ;
#2530=ORIENTED_EDGE ( 'NONE', *, *, #161, .F. ) ;
#2555=CYLINDRICAL_SURFACE ( 'NONE', #2647, 2.499999999999999556 ) ;
#2590=AXIS2_PLACEMENT_3D ( 'NONE', #595, #1331, #2413 ) ;
#2593=AXIS2_PLACEMENT_3D ( 'NONE', #1415, #723, #915 ) ;
#2612=EDGE_CURVE ( 'NONE', #2199, #2182, #1608, .T. ) ;
#2624=CARTESIAN_POINT ( 'NONE',  ( -2.499999999999999556, 3.061616997868382648E-16, 18.00000000000000355 ) ) ;
#2643=ORIENTED_EDGE ( 'NONE', *, *, #2213, .F. ) ;
#2647=AXIS2_PLACEMENT_3D ( 'NONE', #252, #1760, #561 ) ;
#2651=( GEOMETRIC_REPRESENTATION_CONTEXT ( 3 ) GLOBAL_UNCERTAINTY_ASSIGNED_CONTEXT ( ( #1761 ) ) GLOBAL_UNIT_ASSIGNED_CONTEXT ( ( #2666, #3148, #2817 ) ) REPRESENTATION_CONTEXT ( 'NONE', 'WORKASPACE' ) );
#2659=EDGE_LOOP ( 'NONE', ( #567, #2140, #1257, #560 ) ) ;
#2660=DIRECTION ( 'NONE',  ( 1.000000000000000000, 0.000000000000000000, 0.000000000000000000 ) ) ;
#2664=EDGE_LOOP ( 'NONE', ( #376, #1610, #928, #3200 ) ) ;
#2666=( LENGTH_UNIT ( ) NAMED_UNIT ( * ) SI_UNIT ( .MILLI., .METRE. ) );
#2673=ORIENTED_EDGE ( 'NONE', *, *, #303, .F. ) ;
#2678=VECTOR ( 'NONE', #1025, 1000.000000000000000 ) ;
#2684=AXIS2_PLACEMENT_3D ( 'NONE', #790, #1315, #2330 ) ;
#2687=CYLINDRICAL_SURFACE ( 'NONE', #138, 7.500000000000000888 ) ;
#2693=DIRECTION ( 'NONE',  ( -0.000000000000000000, -0.000000000000000000, 1.000000000000000000 ) ) ;
#2706=FACE_OUTER_BOUND ( 'NONE', #563, .T. ) ;
#2708=VERTEX_POINT ( 'NONE', #1122 ) ;
#2712=EDGE_CURVE ( 'NONE', #694, #2708, #2137, .T. ) ;
#2723=ORIENTED_EDGE ( 'NONE', *, *, #558, .T. ) ;
#2729=CARTESIAN_POINT ( 'NONE',  ( 7.500000000000000000, 9.184850993605147944E-16, 18.00000000000000355 ) ) ;
#2731=DIRECTION ( 'NONE',  ( -0.000000000000000000, -0.000000000000000000, -1.000000000000000000 ) ) ;
#2749=EDGE_CURVE ( 'NONE', #1883, #439, #2383, .T. ) ;
#2752=AXIS2_PLACEMENT_3D ( 'NONE', #2289, #676, #3202 ) ;
#2755=DIRECTION ( 'NONE',  ( 1.000000000000000000, 0.000000000000000000, 0.000000000000000000 ) ) ;
#2757=CARTESIAN_POINT ( 'NONE',  ( 0.000000000000000000, 0.000000000000000000, 10.00000000000000000 ) ) ;
#2766=PRODUCT_CONTEXT ( 'NONE', #1465, 'mechanical' ) ;
#2781=EDGE_CURVE ( 'NONE', #2412, #1810, #3121, .T. ) ;
#2784=DIRECTION ( 'NONE',  ( -0.000000000000000000, -0.000000000000000000, -1.000000000000000000 ) ) ;
#2795=AXIS2_PLACEMENT_3D ( 'NONE', #696, #3003, #725 ) ;
#2801=DIRECTION ( 'NONE',  ( 1.000000000000000000, 0.000000000000000000, 0.000000000000000000 ) ) ;
#2803=PLANE ( 'NONE',  #3163 ) ;
#2817=( NAMED_UNIT ( * ) SI_UNIT ( $, .STERADIAN. ) SOLID_ANGLE_UNIT ( ) );
#2822=EDGE_CURVE ( 'NONE', #1087, #3085, #1793, .T. ) ;
#2835=FILL_AREA_STYLE_COLOUR ( '', #2909 ) ;
#2840=EDGE_CURVE ( 'NONE', #342, #3085, #1449, .T. ) ;
#2843=LINE ( 'NONE', #1785, #630 ) ;
#2855=ADVANCED_FACE ( 'NONE', ( #2428 ), #153, .F. ) ;
#2857=CARTESIAN_POINT ( 'NONE',  ( -5.000000000000000000, 30.00000000000000000, -21.62277660168378901 ) ) ;
#2868=EDGE_CURVE ( 'NONE', #1046, #2883, #3228, .T. ) ;
#2870=VERTEX_POINT ( 'NONE', #3239 ) ;
#2883=VERTEX_POINT ( 'NONE', #2497 ) ;
#2889=CARTESIAN_POINT ( 'NONE',  ( 0.000000000000000000, 0.000000000000000000, 10.00000000000000000 ) ) ;
#2904=CIRCLE ( 'NONE', #1162, 7.500000000000000000 ) ;
#2909=COLOUR_RGB ( '',0.8941176470588234615, 0.8941176470588234615, 0.8941176470588234615 ) ;
#2917=ORIENTED_EDGE ( 'NONE', *, *, #1884, .F. ) ;
#2928=ADVANCED_FACE ( 'NONE', ( #1030 ), #2555, .F. ) ;
#2931=EDGE_LOOP ( 'NONE', ( #2480, #2446, #2723, #2917 ) ) ;
#2933=FACE_OUTER_BOUND ( 'NONE', #2931, .T. ) ;
#2936=CARTESIAN_POINT ( 'NONE',  ( 0.000000000000000000, 30.00000000000000000, 10.00000000000000000 ) ) ;
#2946=VECTOR ( 'NONE', #2119, 1000.000000000000000 ) ;
#2956=DIRECTION ( 'NONE',  ( 0.000000000000000000, 0.000000000000000000, 1.000000000000000000 ) ) ;
#2960=CARTESIAN_POINT ( 'NONE',  ( 0.000000000000000000, 0.000000000000000000, 18.00000000000000355 ) ) ;
#2973=DIRECTION ( 'NONE',  ( -0.000000000000000000, -0.000000000000000000, 1.000000000000000000 ) ) ;
#2975=FACE_BOUND ( 'NONE', #2136, .T. ) ;
#2976=DIRECTION ( 'NONE',  ( 0.000000000000000000, 0.000000000000000000, 1.000000000000000000 ) ) ;
#2977=CARTESIAN_POINT ( 'NONE',  ( 0.000000000000000000, 0.000000000000000000, 18.00000000000000355 ) ) ;
#2987=DIRECTION ( 'NONE',  ( 0.000000000000000000, 0.000000000000000000, 1.000000000000000000 ) ) ;
#2988=EDGE_CURVE ( 'NONE', #2883, #1087, #1639, .T. ) ;
#2990=CARTESIAN_POINT ( 'NONE',  ( 0.000000000000000000, 30.00000000000000000, 18.00000000000000355 ) ) ;
#2997=CIRCLE ( 'NONE', #2684, 4.999999999999999112 ) ;
#3003=DIRECTION ( 'NONE',  ( 0.000000000000000000, 0.000000000000000000, 1.000000000000000000 ) ) ;
#3006=DIRECTION ( 'NONE',  ( 1.000000000000000000, 0.000000000000000000, 0.000000000000000000 ) ) ;
#3007=CIRCLE ( 'NONE', #1424, 7.500000000000000000 ) ;
#3016=SHAPE_DEFINITION_REPRESENTATION ( #886, #1236 ) ;
#3022=PLANE ( 'NONE',  #2525 ) ;
#3031=LINE ( 'NONE', #1016, #1902 ) ;
#3048=UNCERTAINTY_MEASURE_WITH_UNIT (LENGTH_MEASURE( 1.000000000000000082E-05 ), #30, 'distance_accuracy_value', 'NONE');
#3051=( NAMED_UNIT ( * ) PLANE_ANGLE_UNIT ( ) SI_UNIT ( $, .RADIAN. ) );
#3056=( NAMED_UNIT ( * ) SI_UNIT ( $, .STERADIAN. ) SOLID_ANGLE_UNIT ( ) );
#3057=PRODUCT_DEFINITION ( 'UNKNOWN', '', #856, #1001 ) ;
#3059=VECTOR ( 'NONE', #1514, 1000.000000000000000 ) ;
#3075=CARTESIAN_POINT ( 'NONE',  ( 0.000000000000000000, 0.000000000000000000, 0.000000000000000000 ) ) ;
#3085=VERTEX_POINT ( 'NONE', #1894 ) ;
#3093=EDGE_CURVE ( 'NONE', #2199, #694, #742, .T. ) ;
#3107=CIRCLE ( 'NONE', #248, 2.500000000000000000 ) ;
#3108=FACE_OUTER_BOUND ( 'NONE', #1963, .T. ) ;
#3115=DIRECTION ( 'NONE',  ( 1.000000000000000000, 0.000000000000000000, 0.000000000000000000 ) ) ;
#3119=CIRCLE ( 'NONE', #583, 7.500000000000000000 ) ;
#3121=CIRCLE ( 'NONE', #1375, 4.999999999999998224 ) ;
#3130=VERTEX_POINT ( 'NONE', #71 ) ;
#3141=ADVANCED_FACE ( 'NONE', ( #2933 ), #2197, .T. ) ;
#3144=LINE ( 'NONE', #60, #2946 ) ;
#3148=( NAMED_UNIT ( * ) PLANE_ANGLE_UNIT ( ) SI_UNIT ( $, .RADIAN. ) );
#3157=ORIENTED_EDGE ( 'NONE', *, *, #2125, .T. ) ;
#3159=AXIS2_PLACEMENT_3D ( 'NONE', #2960, #2976, #3006 ) ;
#3163=AXIS2_PLACEMENT_3D ( 'NONE', #1797, #989, #2005 ) ;
#3173=AXIS2_PLACEMENT_3D ( 'NONE', #1031, #789, #2801 ) ;
#3179=CARTESIAN_POINT ( 'NONE',  ( 0.000000000000000000, 0.000000000000000000, 18.00000000000000355 ) ) ;
#3180=AXIS2_PLACEMENT_3D ( 'NONE', #1929, #2693, #1966 ) ;
#3189=EDGE_LOOP ( 'NONE', ( #865, #1803, #2292, #1180 ) ) ;
#3192=DIRECTION ( 'NONE',  ( 1.000000000000000000, 0.000000000000000000, 0.000000000000000000 ) ) ;
#3200=ORIENTED_EDGE ( 'NONE', *, *, #3241, .T. ) ;
#3202=DIRECTION ( 'NONE',  ( -1.000000000000000000, 0.000000000000000000, 0.000000000000000000 ) ) ;
#3207=FACE_OUTER_BOUND ( 'NONE', #933, .T. ) ;
#3209=FACE_OUTER_BOUND ( 'NONE', #352, .T. ) ;
#3214=VERTEX_POINT ( 'NONE', #1022 ) ;
#3226=CARTESIAN_POINT ( 'NONE',  ( 0.000000000000000000, 0.000000000000000000, 18.00000000000000355 ) ) ;
#3228=CIRCLE ( 'NONE', #2014, 7.500000000000000888 ) ;
#3232=DIRECTION ( 'NONE',  ( 0.000000000000000000, 0.000000000000000000, 1.000000000000000000 ) ) ;
#3239=CARTESIAN_POINT ( 'NONE',  ( -7.500000000000000000, 0.000000000000000000, 18.00000000000000355 ) ) ;
#3241=EDGE_CURVE ( 'NONE', #2195, #870, #2493, .T. ) ;
#3243=DIRECTION ( 'NONE',  ( 0.000000000000000000, 0.000000000000000000, 1.000000000000000000 ) ) ;
#3256=PLANE ( 'NONE',  #1212 ) ;
#3258=ADVANCED_FACE ( 'NONE', ( #2478 ), #1726, .T. ) ;
#3259=AXIS2_PLACEMENT_3D ( 'NONE', #1208, #3232, #1051 ) ;
#3268=LINE ( 'NONE', #997, #1248 ) ;
#3273=FACE_OUTER_BOUND ( 'NONE', #2460, .T. ) ;
#3294=COLOUR_RGB('Sky Blue',0.24,0.69,0.87);
#3295=FILL_AREA_STYLE_COLOUR('',#3294);
#3296=FILL_AREA_STYLE('',(#3295));
#3297=SURFACE_STYLE_FILL_AREA(#3296);
#3298=SURFACE_SIDE_STYLE('',(#3297));
#3299=SURFACE_STYLE_USAGE(.BOTH.,#3298);
#3300=PRESENTATION_STYLE_ASSIGNMENT((#3299));
ENDSEC;
END-ISO-10303-21;
